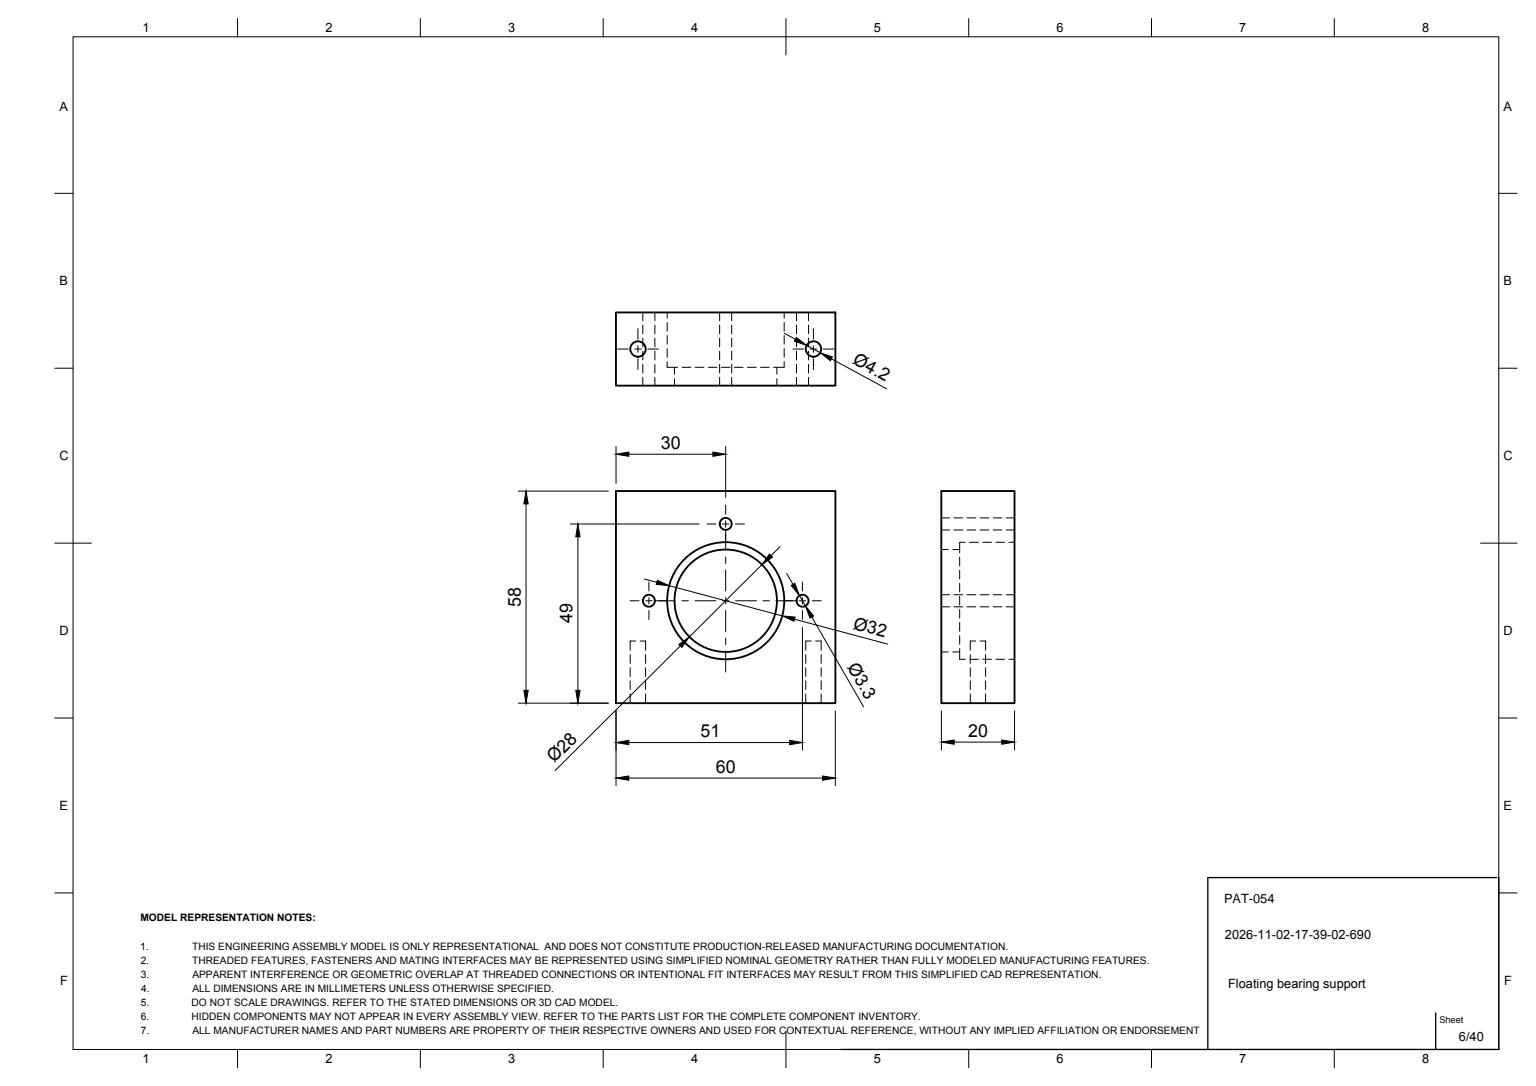
ISO-10303-21;
HEADER;
/* Generated by software containing ST-Developer
 * from STEP Tools, Inc. (www.steptools.com) 
 */

FILE_DESCRIPTION(
/* description */ ('PAT-054'),
/* implementation_level */ '2;1');

FILE_NAME(
/* name */ 'Floating bearing support.step',
/* time_stamp */ '2026-10-29T16:38:13-07:00',
/* author */ (''),
/* organization */ (''),
/* preprocessor_version */ 'ST-DEVELOPER v20.2',
/* originating_system */ 'Autodesk Translation Framework v15.17.0.0',
/* authorisation */ '');

FILE_SCHEMA (('AUTOMOTIVE_DESIGN { 1 0 10303 214 3 1 1 }'));
ENDSEC;

DATA;
#10=MECHANICAL_DESIGN_GEOMETRIC_PRESENTATION_REPRESENTATION('',(#901),#33981);
#813=SHAPE_REPRESENTATION_RELATIONSHIP('SRR','None',#34186,#857);
#857=ADVANCED_BREP_SHAPE_REPRESENTATION('',(#960),#33934);
#901=STYLED_ITEM('',(#34517),#960);
#960=MANIFOLD_SOLID_BREP('Body1',#13012);
#1064=FACE_BOUND('',#2399,.T.);
#1065=FACE_BOUND('',#2407,.T.);
#1066=FACE_BOUND('',#2408,.T.);
#1067=FACE_BOUND('',#2409,.T.);
#1068=FACE_BOUND('',#2410,.T.);
#1069=FACE_BOUND('',#2413,.T.);
#1070=FACE_BOUND('',#2414,.T.);
#1071=FACE_BOUND('',#2415,.T.);
#1072=FACE_BOUND('',#2416,.T.);
#1073=FACE_BOUND('',#2419,.T.);
#1074=FACE_BOUND('',#2420,.T.);
#1244=PLANE('',#13676);
#1245=PLANE('',#13683);
#1246=PLANE('',#13687);
#1247=PLANE('',#13688);
#1248=PLANE('',#13689);
#1249=PLANE('',#13690);
#1250=PLANE('',#13691);
#1251=PLANE('',#13692);
#1252=PLANE('',#13693);
#1619=FACE_OUTER_BOUND('',#2394,.T.);
#1620=FACE_OUTER_BOUND('',#2395,.T.);
#1621=FACE_OUTER_BOUND('',#2396,.T.);
#1622=FACE_OUTER_BOUND('',#2397,.T.);
#1623=FACE_OUTER_BOUND('',#2398,.T.);
#1624=FACE_OUTER_BOUND('',#2400,.T.);
#1625=FACE_OUTER_BOUND('',#2401,.T.);
#1626=FACE_OUTER_BOUND('',#2402,.T.);
#1627=FACE_OUTER_BOUND('',#2403,.T.);
#1628=FACE_OUTER_BOUND('',#2404,.T.);
#1629=FACE_OUTER_BOUND('',#2405,.T.);
#1630=FACE_OUTER_BOUND('',#2406,.T.);
#1631=FACE_OUTER_BOUND('',#2411,.T.);
#1632=FACE_OUTER_BOUND('',#2412,.T.);
#1633=FACE_OUTER_BOUND('',#2417,.T.);
#1634=FACE_OUTER_BOUND('',#2418,.T.);
#2394=EDGE_LOOP('',(#8705,#8706,#8707,#8708));
#2395=EDGE_LOOP('',(#8709,#8710,#8711,#8712));
#2396=EDGE_LOOP('',(#8713,#8714,#8715,#8716));
#2397=EDGE_LOOP('',(#8717,#8718,#8719,#8720));
#2398=EDGE_LOOP('',(#8721));
#2399=EDGE_LOOP('',(#8722));
#2400=EDGE_LOOP('',(#8723,#8724,#8725,#8726));
#2401=EDGE_LOOP('',(#8727,#8728,#8729,#8730));
#2402=EDGE_LOOP('',(#8731));
#2403=EDGE_LOOP('',(#8732,#8733,#8734,#8735));
#2404=EDGE_LOOP('',(#8736));
#2405=EDGE_LOOP('',(#8737,#8738,#8739,#8740));
#2406=EDGE_LOOP('',(#8741,#8742,#8743,#8744));
#2407=EDGE_LOOP('',(#8745));
#2408=EDGE_LOOP('',(#8746));
#2409=EDGE_LOOP('',(#8747));
#2410=EDGE_LOOP('',(#8748));
#2411=EDGE_LOOP('',(#8749,#8750,#8751,#8752));
#2412=EDGE_LOOP('',(#8753,#8754,#8755,#8756));
#2413=EDGE_LOOP('',(#8757));
#2414=EDGE_LOOP('',(#8758));
#2415=EDGE_LOOP('',(#8759));
#2416=EDGE_LOOP('',(#8760));
#2417=EDGE_LOOP('',(#8761,#8762,#8763,#8764));
#2418=EDGE_LOOP('',(#8765,#8766,#8767,#8768));
#2419=EDGE_LOOP('',(#8769));
#2420=EDGE_LOOP('',(#8770));
#3289=LINE('',#18719,#4223);
#3290=LINE('',#18725,#4224);
#3291=LINE('',#18731,#4225);
#3292=LINE('',#18737,#4226);
#3293=LINE('',#18744,#4227);
#3294=LINE('',#18750,#4228);
#3295=LINE('',#18757,#4229);
#3296=LINE('',#18763,#4230);
#3297=LINE('',#18765,#4231);
#3298=LINE('',#18767,#4232);
#3299=LINE('',#18768,#4233);
#3300=LINE('',#18771,#4234);
#3301=LINE('',#18773,#4235);
#3302=LINE('',#18774,#4236);
#3303=LINE('',#18777,#4237);
#3304=LINE('',#18779,#4238);
#3305=LINE('',#18780,#4239);
#3306=LINE('',#18782,#4240);
#3307=LINE('',#18783,#4241);
#4223=VECTOR('',#15156,0.165);
#4224=VECTOR('',#15163,0.165);
#4225=VECTOR('',#15170,0.165);
#4226=VECTOR('',#15177,1.6);
#4227=VECTOR('',#15186,1.4);
#4228=VECTOR('',#15193,0.21);
#4229=VECTOR('',#15202,0.21);
#4230=VECTOR('',#15209,1.);
#4231=VECTOR('',#15210,1.);
#4232=VECTOR('',#15211,1.);
#4233=VECTOR('',#15212,1.);
#4234=VECTOR('',#15215,1.);
#4235=VECTOR('',#15216,1.);
#4236=VECTOR('',#15217,1.);
#4237=VECTOR('',#15220,1.);
#4238=VECTOR('',#15221,1.);
#4239=VECTOR('',#15222,1.);
#4240=VECTOR('',#15225,1.);
#4241=VECTOR('',#15226,1.);
#5161=CIRCLE('',#13665,0.165);
#5162=CIRCLE('',#13666,0.165);
#5163=CIRCLE('',#13668,0.165);
#5164=CIRCLE('',#13669,0.165);
#5165=CIRCLE('',#13671,0.165);
#5166=CIRCLE('',#13672,0.165);
#5167=CIRCLE('',#13674,1.6);
#5168=CIRCLE('',#13675,1.6);
#5169=CIRCLE('',#13677,1.4);
#5170=CIRCLE('',#13679,1.4);
#5171=CIRCLE('',#13681,0.21);
#5172=CIRCLE('',#13682,0.21);
#5173=CIRCLE('',#13685,0.21);
#5174=CIRCLE('',#13686,0.21);
#5642=VERTEX_POINT('',#18716);
#5643=VERTEX_POINT('',#18718);
#5644=VERTEX_POINT('',#18722);
#5645=VERTEX_POINT('',#18724);
#5646=VERTEX_POINT('',#18728);
#5647=VERTEX_POINT('',#18730);
#5648=VERTEX_POINT('',#18734);
#5649=VERTEX_POINT('',#18736);
#5650=VERTEX_POINT('',#18740);
#5651=VERTEX_POINT('',#18743);
#5652=VERTEX_POINT('',#18747);
#5653=VERTEX_POINT('',#18749);
#5654=VERTEX_POINT('',#18754);
#5655=VERTEX_POINT('',#18756);
#5656=VERTEX_POINT('',#18761);
#5657=VERTEX_POINT('',#18762);
#5658=VERTEX_POINT('',#18764);
#5659=VERTEX_POINT('',#18766);
#5660=VERTEX_POINT('',#18770);
#5661=VERTEX_POINT('',#18772);
#5662=VERTEX_POINT('',#18776);
#5663=VERTEX_POINT('',#18778);
#6852=EDGE_CURVE('',#5642,#5642,#5161,.T.);
#6853=EDGE_CURVE('',#5642,#5643,#3289,.T.);
#6854=EDGE_CURVE('',#5643,#5643,#5162,.T.);
#6855=EDGE_CURVE('',#5644,#5644,#5163,.T.);
#6856=EDGE_CURVE('',#5644,#5645,#3290,.T.);
#6857=EDGE_CURVE('',#5645,#5645,#5164,.T.);
#6858=EDGE_CURVE('',#5646,#5646,#5165,.T.);
#6859=EDGE_CURVE('',#5646,#5647,#3291,.T.);
#6860=EDGE_CURVE('',#5647,#5647,#5166,.T.);
#6861=EDGE_CURVE('',#5648,#5648,#5167,.T.);
#6862=EDGE_CURVE('',#5648,#5649,#3292,.T.);
#6863=EDGE_CURVE('',#5649,#5649,#5168,.T.);
#6864=EDGE_CURVE('',#5650,#5650,#5169,.T.);
#6865=EDGE_CURVE('',#5650,#5651,#3293,.T.);
#6866=EDGE_CURVE('',#5651,#5651,#5170,.T.);
#6867=EDGE_CURVE('',#5652,#5652,#5171,.T.);
#6868=EDGE_CURVE('',#5652,#5653,#3294,.T.);
#6869=EDGE_CURVE('',#5653,#5653,#5172,.T.);
#6870=EDGE_CURVE('',#5654,#5654,#5173,.T.);
#6871=EDGE_CURVE('',#5654,#5655,#3295,.T.);
#6872=EDGE_CURVE('',#5655,#5655,#5174,.T.);
#6873=EDGE_CURVE('',#5656,#5657,#3296,.T.);
#6874=EDGE_CURVE('',#5657,#5658,#3297,.T.);
#6875=EDGE_CURVE('',#5659,#5658,#3298,.T.);
#6876=EDGE_CURVE('',#5656,#5659,#3299,.T.);
#6877=EDGE_CURVE('',#5660,#5656,#3300,.T.);
#6878=EDGE_CURVE('',#5661,#5659,#3301,.T.);
#6879=EDGE_CURVE('',#5660,#5661,#3302,.T.);
#6880=EDGE_CURVE('',#5662,#5660,#3303,.T.);
#6881=EDGE_CURVE('',#5663,#5661,#3304,.T.);
#6882=EDGE_CURVE('',#5662,#5663,#3305,.T.);
#6883=EDGE_CURVE('',#5657,#5662,#3306,.T.);
#6884=EDGE_CURVE('',#5658,#5663,#3307,.T.);
#8705=ORIENTED_EDGE('',*,*,#6852,.F.);
#8706=ORIENTED_EDGE('',*,*,#6853,.T.);
#8707=ORIENTED_EDGE('',*,*,#6854,.F.);
#8708=ORIENTED_EDGE('',*,*,#6853,.F.);
#8709=ORIENTED_EDGE('',*,*,#6855,.F.);
#8710=ORIENTED_EDGE('',*,*,#6856,.T.);
#8711=ORIENTED_EDGE('',*,*,#6857,.F.);
#8712=ORIENTED_EDGE('',*,*,#6856,.F.);
#8713=ORIENTED_EDGE('',*,*,#6858,.F.);
#8714=ORIENTED_EDGE('',*,*,#6859,.T.);
#8715=ORIENTED_EDGE('',*,*,#6860,.F.);
#8716=ORIENTED_EDGE('',*,*,#6859,.F.);
#8717=ORIENTED_EDGE('',*,*,#6861,.F.);
#8718=ORIENTED_EDGE('',*,*,#6862,.T.);
#8719=ORIENTED_EDGE('',*,*,#6863,.T.);
#8720=ORIENTED_EDGE('',*,*,#6862,.F.);
#8721=ORIENTED_EDGE('',*,*,#6863,.F.);
#8722=ORIENTED_EDGE('',*,*,#6864,.F.);
#8723=ORIENTED_EDGE('',*,*,#6864,.T.);
#8724=ORIENTED_EDGE('',*,*,#6865,.T.);
#8725=ORIENTED_EDGE('',*,*,#6866,.F.);
#8726=ORIENTED_EDGE('',*,*,#6865,.F.);
#8727=ORIENTED_EDGE('',*,*,#6867,.F.);
#8728=ORIENTED_EDGE('',*,*,#6868,.T.);
#8729=ORIENTED_EDGE('',*,*,#6869,.T.);
#8730=ORIENTED_EDGE('',*,*,#6868,.F.);
#8731=ORIENTED_EDGE('',*,*,#6869,.F.);
#8732=ORIENTED_EDGE('',*,*,#6870,.F.);
#8733=ORIENTED_EDGE('',*,*,#6871,.T.);
#8734=ORIENTED_EDGE('',*,*,#6872,.T.);
#8735=ORIENTED_EDGE('',*,*,#6871,.F.);
#8736=ORIENTED_EDGE('',*,*,#6872,.F.);
#8737=ORIENTED_EDGE('',*,*,#6873,.T.);
#8738=ORIENTED_EDGE('',*,*,#6874,.T.);
#8739=ORIENTED_EDGE('',*,*,#6875,.F.);
#8740=ORIENTED_EDGE('',*,*,#6876,.F.);
#8741=ORIENTED_EDGE('',*,*,#6877,.T.);
#8742=ORIENTED_EDGE('',*,*,#6876,.T.);
#8743=ORIENTED_EDGE('',*,*,#6878,.F.);
#8744=ORIENTED_EDGE('',*,*,#6879,.F.);
#8745=ORIENTED_EDGE('',*,*,#6854,.T.);
#8746=ORIENTED_EDGE('',*,*,#6857,.T.);
#8747=ORIENTED_EDGE('',*,*,#6860,.T.);
#8748=ORIENTED_EDGE('',*,*,#6866,.T.);
#8749=ORIENTED_EDGE('',*,*,#6880,.T.);
#8750=ORIENTED_EDGE('',*,*,#6879,.T.);
#8751=ORIENTED_EDGE('',*,*,#6881,.F.);
#8752=ORIENTED_EDGE('',*,*,#6882,.F.);
#8753=ORIENTED_EDGE('',*,*,#6883,.T.);
#8754=ORIENTED_EDGE('',*,*,#6882,.T.);
#8755=ORIENTED_EDGE('',*,*,#6884,.F.);
#8756=ORIENTED_EDGE('',*,*,#6874,.F.);
#8757=ORIENTED_EDGE('',*,*,#6852,.T.);
#8758=ORIENTED_EDGE('',*,*,#6855,.T.);
#8759=ORIENTED_EDGE('',*,*,#6858,.T.);
#8760=ORIENTED_EDGE('',*,*,#6861,.T.);
#8761=ORIENTED_EDGE('',*,*,#6884,.T.);
#8762=ORIENTED_EDGE('',*,*,#6881,.T.);
#8763=ORIENTED_EDGE('',*,*,#6878,.T.);
#8764=ORIENTED_EDGE('',*,*,#6875,.T.);
#8765=ORIENTED_EDGE('',*,*,#6883,.F.);
#8766=ORIENTED_EDGE('',*,*,#6873,.F.);
#8767=ORIENTED_EDGE('',*,*,#6877,.F.);
#8768=ORIENTED_EDGE('',*,*,#6880,.F.);
#8769=ORIENTED_EDGE('',*,*,#6867,.T.);
#8770=ORIENTED_EDGE('',*,*,#6870,.T.);
#12007=CYLINDRICAL_SURFACE('',#13664,0.165);
#12008=CYLINDRICAL_SURFACE('',#13667,0.165);
#12009=CYLINDRICAL_SURFACE('',#13670,0.165);
#12010=CYLINDRICAL_SURFACE('',#13673,1.6);
#12011=CYLINDRICAL_SURFACE('',#13678,1.4);
#12012=CYLINDRICAL_SURFACE('',#13680,0.21);
#12013=CYLINDRICAL_SURFACE('',#13684,0.21);
#12331=ADVANCED_FACE('',(#1619),#12007,.F.);
#12332=ADVANCED_FACE('',(#1620),#12008,.F.);
#12333=ADVANCED_FACE('',(#1621),#12009,.F.);
#12334=ADVANCED_FACE('',(#1622),#12010,.F.);
#12335=ADVANCED_FACE('',(#1623,#1064),#1244,.F.);
#12336=ADVANCED_FACE('',(#1624),#12011,.F.);
#12337=ADVANCED_FACE('',(#1625),#12012,.F.);
#12338=ADVANCED_FACE('',(#1626),#1245,.F.);
#12339=ADVANCED_FACE('',(#1627),#12013,.F.);
#12340=ADVANCED_FACE('',(#1628),#1246,.F.);
#12341=ADVANCED_FACE('',(#1629),#1247,.T.);
#12342=ADVANCED_FACE('',(#1630,#1065,#1066,#1067,#1068),#1248,.T.);
#12343=ADVANCED_FACE('',(#1631),#1249,.T.);
#12344=ADVANCED_FACE('',(#1632,#1069,#1070,#1071,#1072),#1250,.T.);
#12345=ADVANCED_FACE('',(#1633),#1251,.T.);
#12346=ADVANCED_FACE('',(#1634,#1073,#1074),#1252,.F.);
#13012=CLOSED_SHELL('',(#12331,#12332,#12333,#12334,#12335,#12336,#12337,
#12338,#12339,#12340,#12341,#12342,#12343,#12344,#12345,#12346));
#13663=AXIS2_PLACEMENT_3D('',#18714,#15150,#15151);
#13664=AXIS2_PLACEMENT_3D('',#18715,#15152,#15153);
#13665=AXIS2_PLACEMENT_3D('',#18717,#15154,#15155);
#13666=AXIS2_PLACEMENT_3D('',#18720,#15157,#15158);
#13667=AXIS2_PLACEMENT_3D('',#18721,#15159,#15160);
#13668=AXIS2_PLACEMENT_3D('',#18723,#15161,#15162);
#13669=AXIS2_PLACEMENT_3D('',#18726,#15164,#15165);
#13670=AXIS2_PLACEMENT_3D('',#18727,#15166,#15167);
#13671=AXIS2_PLACEMENT_3D('',#18729,#15168,#15169);
#13672=AXIS2_PLACEMENT_3D('',#18732,#15171,#15172);
#13673=AXIS2_PLACEMENT_3D('',#18733,#15173,#15174);
#13674=AXIS2_PLACEMENT_3D('',#18735,#15175,#15176);
#13675=AXIS2_PLACEMENT_3D('',#18738,#15178,#15179);
#13676=AXIS2_PLACEMENT_3D('',#18739,#15180,#15181);
#13677=AXIS2_PLACEMENT_3D('',#18741,#15182,#15183);
#13678=AXIS2_PLACEMENT_3D('',#18742,#15184,#15185);
#13679=AXIS2_PLACEMENT_3D('',#18745,#15187,#15188);
#13680=AXIS2_PLACEMENT_3D('',#18746,#15189,#15190);
#13681=AXIS2_PLACEMENT_3D('',#18748,#15191,#15192);
#13682=AXIS2_PLACEMENT_3D('',#18751,#15194,#15195);
#13683=AXIS2_PLACEMENT_3D('',#18752,#15196,#15197);
#13684=AXIS2_PLACEMENT_3D('',#18753,#15198,#15199);
#13685=AXIS2_PLACEMENT_3D('',#18755,#15200,#15201);
#13686=AXIS2_PLACEMENT_3D('',#18758,#15203,#15204);
#13687=AXIS2_PLACEMENT_3D('',#18759,#15205,#15206);
#13688=AXIS2_PLACEMENT_3D('',#18760,#15207,#15208);
#13689=AXIS2_PLACEMENT_3D('',#18769,#15213,#15214);
#13690=AXIS2_PLACEMENT_3D('',#18775,#15218,#15219);
#13691=AXIS2_PLACEMENT_3D('',#18781,#15223,#15224);
#13692=AXIS2_PLACEMENT_3D('',#18784,#15227,#15228);
#13693=AXIS2_PLACEMENT_3D('',#18785,#15229,#15230);
#15150=DIRECTION('axis',(0.,0.,1.));
#15151=DIRECTION('refdir',(1.,0.,0.));
#15152=DIRECTION('center_axis',(1.,0.,0.));
#15153=DIRECTION('ref_axis',(0.,0.,-1.));
#15154=DIRECTION('center_axis',(1.,0.,0.));
#15155=DIRECTION('ref_axis',(0.,0.,-1.));
#15156=DIRECTION('',(1.,0.,0.));
#15157=DIRECTION('center_axis',(-1.,0.,0.));
#15158=DIRECTION('ref_axis',(0.,0.,-1.));
#15159=DIRECTION('center_axis',(1.,0.,0.));
#15160=DIRECTION('ref_axis',(0.,0.,-1.));
#15161=DIRECTION('center_axis',(1.,0.,0.));
#15162=DIRECTION('ref_axis',(0.,0.,-1.));
#15163=DIRECTION('',(1.,0.,0.));
#15164=DIRECTION('center_axis',(-1.,0.,0.));
#15165=DIRECTION('ref_axis',(0.,0.,-1.));
#15166=DIRECTION('center_axis',(1.,0.,0.));
#15167=DIRECTION('ref_axis',(0.,0.,-1.));
#15168=DIRECTION('center_axis',(1.,0.,0.));
#15169=DIRECTION('ref_axis',(0.,0.,-1.));
#15170=DIRECTION('',(1.,0.,0.));
#15171=DIRECTION('center_axis',(-1.,0.,0.));
#15172=DIRECTION('ref_axis',(0.,0.,-1.));
#15173=DIRECTION('center_axis',(1.,0.,0.));
#15174=DIRECTION('ref_axis',(0.,0.,-1.));
#15175=DIRECTION('center_axis',(1.,0.,0.));
#15176=DIRECTION('ref_axis',(0.,0.,-1.));
#15177=DIRECTION('',(1.,0.,0.));
#15178=DIRECTION('center_axis',(1.,0.,0.));
#15179=DIRECTION('ref_axis',(0.,0.,-1.));
#15180=DIRECTION('center_axis',(1.,0.,0.));
#15181=DIRECTION('ref_axis',(0.,0.,-1.));
#15182=DIRECTION('center_axis',(-1.,0.,0.));
#15183=DIRECTION('ref_axis',(0.,0.,-1.));
#15184=DIRECTION('center_axis',(1.,0.,0.));
#15185=DIRECTION('ref_axis',(0.,0.,-1.));
#15186=DIRECTION('',(1.,0.,0.));
#15187=DIRECTION('center_axis',(-1.,0.,0.));
#15188=DIRECTION('ref_axis',(0.,0.,-1.));
#15189=DIRECTION('center_axis',(0.,0.,1.));
#15190=DIRECTION('ref_axis',(1.,0.,0.));
#15191=DIRECTION('center_axis',(0.,0.,1.));
#15192=DIRECTION('ref_axis',(1.,0.,0.));
#15193=DIRECTION('',(0.,0.,1.));
#15194=DIRECTION('center_axis',(0.,0.,1.));
#15195=DIRECTION('ref_axis',(1.,0.,0.));
#15196=DIRECTION('center_axis',(0.,0.,1.));
#15197=DIRECTION('ref_axis',(1.,0.,0.));
#15198=DIRECTION('center_axis',(0.,0.,1.));
#15199=DIRECTION('ref_axis',(1.,0.,0.));
#15200=DIRECTION('center_axis',(0.,0.,1.));
#15201=DIRECTION('ref_axis',(1.,0.,0.));
#15202=DIRECTION('',(0.,0.,1.));
#15203=DIRECTION('center_axis',(0.,0.,1.));
#15204=DIRECTION('ref_axis',(1.,0.,0.));
#15205=DIRECTION('center_axis',(0.,0.,1.));
#15206=DIRECTION('ref_axis',(1.,0.,0.));
#15207=DIRECTION('center_axis',(0.,1.,0.));
#15208=DIRECTION('ref_axis',(-1.,0.,0.));
#15209=DIRECTION('',(-1.,0.,0.));
#15210=DIRECTION('',(0.,0.,1.));
#15211=DIRECTION('',(-1.,0.,0.));
#15212=DIRECTION('',(0.,0.,1.));
#15213=DIRECTION('center_axis',(1.,0.,0.));
#15214=DIRECTION('ref_axis',(0.,1.,0.));
#15215=DIRECTION('',(0.,1.,0.));
#15216=DIRECTION('',(0.,1.,0.));
#15217=DIRECTION('',(0.,0.,1.));
#15218=DIRECTION('center_axis',(0.,-1.,0.));
#15219=DIRECTION('ref_axis',(1.,0.,0.));
#15220=DIRECTION('',(1.,0.,0.));
#15221=DIRECTION('',(1.,0.,0.));
#15222=DIRECTION('',(0.,0.,1.));
#15223=DIRECTION('center_axis',(-1.,0.,0.));
#15224=DIRECTION('ref_axis',(0.,-1.,0.));
#15225=DIRECTION('',(0.,-1.,0.));
#15226=DIRECTION('',(0.,-1.,0.));
#15227=DIRECTION('center_axis',(0.,0.,1.));
#15228=DIRECTION('ref_axis',(1.,0.,0.));
#15229=DIRECTION('center_axis',(0.,0.,1.));
#15230=DIRECTION('ref_axis',(1.,0.,0.));
#18714=CARTESIAN_POINT('',(0.,0.,0.));
#18715=CARTESIAN_POINT('Origin',(1.9,-2.1,4.));
#18716=CARTESIAN_POINT('',(2.,-2.1,4.165));
#18717=CARTESIAN_POINT('Origin',(2.,-2.1,4.));
#18718=CARTESIAN_POINT('',(4.,-2.1,4.165));
#18719=CARTESIAN_POINT('',(1.9,-2.1,4.165));
#18720=CARTESIAN_POINT('Origin',(4.,-2.1,4.));
#18721=CARTESIAN_POINT('Origin',(1.9,2.1,4.));
#18722=CARTESIAN_POINT('',(2.,2.1,4.165));
#18723=CARTESIAN_POINT('Origin',(2.,2.1,4.));
#18724=CARTESIAN_POINT('',(4.,2.1,4.165));
#18725=CARTESIAN_POINT('',(1.9,2.1,4.165));
#18726=CARTESIAN_POINT('Origin',(4.,2.1,4.));
#18727=CARTESIAN_POINT('Origin',(1.9,0.,6.1));
#18728=CARTESIAN_POINT('',(2.,-2.02066721859313E-17,6.265));
#18729=CARTESIAN_POINT('Origin',(2.,0.,6.1));
#18730=CARTESIAN_POINT('',(4.,2.02066721859313E-17,6.265));
#18731=CARTESIAN_POINT('',(1.9,-2.02066721859313E-17,6.265));
#18732=CARTESIAN_POINT('Origin',(4.,0.,6.1));
#18733=CARTESIAN_POINT('Origin',(1.9,0.,4.));
#18734=CARTESIAN_POINT('',(2.,-1.95943487863577E-16,5.6));
#18735=CARTESIAN_POINT('Origin',(2.,0.,4.));
#18736=CARTESIAN_POINT('',(3.5,-1.95943487863577E-16,5.6));
#18737=CARTESIAN_POINT('',(1.9,-1.95943487863577E-16,5.6));
#18738=CARTESIAN_POINT('Origin',(3.5,0.,4.));
#18739=CARTESIAN_POINT('Origin',(3.5,0.,4.));
#18740=CARTESIAN_POINT('',(3.5,1.71450551880629E-16,5.4));
#18741=CARTESIAN_POINT('Origin',(3.5,0.,4.));
#18742=CARTESIAN_POINT('Origin',(1.9,0.,4.));
#18743=CARTESIAN_POINT('',(4.,1.71450551880629E-16,5.4));
#18744=CARTESIAN_POINT('',(1.9,-1.71450551880629E-16,5.4));
#18745=CARTESIAN_POINT('Origin',(4.,0.,4.));
#18746=CARTESIAN_POINT('Origin',(3.,-2.4,1.1));
#18747=CARTESIAN_POINT('',(2.79,-2.4,1.2));
#18748=CARTESIAN_POINT('Origin',(3.,-2.4,1.2));
#18749=CARTESIAN_POINT('',(2.79,-2.4,2.9));
#18750=CARTESIAN_POINT('',(2.79,-2.4,1.1));
#18751=CARTESIAN_POINT('Origin',(3.,-2.4,2.9));
#18752=CARTESIAN_POINT('Origin',(3.,-2.4,2.9));
#18753=CARTESIAN_POINT('Origin',(3.,2.4,1.1));
#18754=CARTESIAN_POINT('',(2.79,2.4,1.2));
#18755=CARTESIAN_POINT('Origin',(3.,2.4,1.2));
#18756=CARTESIAN_POINT('',(2.79,2.4,2.9));
#18757=CARTESIAN_POINT('',(2.79,2.4,1.1));
#18758=CARTESIAN_POINT('Origin',(3.,2.4,2.9));
#18759=CARTESIAN_POINT('Origin',(3.,2.4,2.9));
#18760=CARTESIAN_POINT('Origin',(4.,3.,1.2));
#18761=CARTESIAN_POINT('',(4.,3.,1.2));
#18762=CARTESIAN_POINT('',(2.,3.,1.2));
#18763=CARTESIAN_POINT('',(4.,3.,1.2));
#18764=CARTESIAN_POINT('',(2.,3.,7.));
#18765=CARTESIAN_POINT('',(2.,3.,1.2));
#18766=CARTESIAN_POINT('',(4.,3.,7.));
#18767=CARTESIAN_POINT('',(4.,3.,7.));
#18768=CARTESIAN_POINT('',(4.,3.,1.2));
#18769=CARTESIAN_POINT('Origin',(4.,-3.,1.2));
#18770=CARTESIAN_POINT('',(4.,-3.,1.2));
#18771=CARTESIAN_POINT('',(4.,-3.,1.2));
#18772=CARTESIAN_POINT('',(4.,-3.,7.));
#18773=CARTESIAN_POINT('',(4.,-3.,7.));
#18774=CARTESIAN_POINT('',(4.,-3.,1.2));
#18775=CARTESIAN_POINT('Origin',(2.,-3.,1.2));
#18776=CARTESIAN_POINT('',(2.,-3.,1.2));
#18777=CARTESIAN_POINT('',(2.,-3.,1.2));
#18778=CARTESIAN_POINT('',(2.,-3.,7.));
#18779=CARTESIAN_POINT('',(2.,-3.,7.));
#18780=CARTESIAN_POINT('',(2.,-3.,1.2));
#18781=CARTESIAN_POINT('Origin',(2.,3.,1.2));
#18782=CARTESIAN_POINT('',(2.,3.,1.2));
#18783=CARTESIAN_POINT('',(2.,3.,7.));
#18784=CARTESIAN_POINT('Origin',(3.,0.,7.));
#18785=CARTESIAN_POINT('Origin',(3.,0.,1.2));
#33882=UNCERTAINTY_MEASURE_WITH_UNIT(LENGTH_MEASURE(0.001),#33982,
'DISTANCE_ACCURACY_VALUE',
'Maximum model space distance between geometric entities at asserted c
onnectivities');
#33929=UNCERTAINTY_MEASURE_WITH_UNIT(LENGTH_MEASURE(0.001),#33982,
'DISTANCE_ACCURACY_VALUE',
'Maximum model space distance between geometric entities at asserted c
onnectivities');
#33934=(
GEOMETRIC_REPRESENTATION_CONTEXT(3)
GLOBAL_UNCERTAINTY_ASSIGNED_CONTEXT((#33882))
GLOBAL_UNIT_ASSIGNED_CONTEXT((#33982,#33984,#33985))
REPRESENTATION_CONTEXT('','3D')
);
#33981=(
GEOMETRIC_REPRESENTATION_CONTEXT(3)
GLOBAL_UNCERTAINTY_ASSIGNED_CONTEXT((#33929))
GLOBAL_UNIT_ASSIGNED_CONTEXT((#33982,#33984,#33985))
REPRESENTATION_CONTEXT('','3D')
);
#33982=(
LENGTH_UNIT()
NAMED_UNIT(*)
SI_UNIT(.CENTI.,.METRE.)
);
#33984=(
NAMED_UNIT(*)
PLANE_ANGLE_UNIT()
SI_UNIT($,.RADIAN.)
);
#33985=(
NAMED_UNIT(*)
SI_UNIT($,.STERADIAN.)
SOLID_ANGLE_UNIT()
);
#33990=SHAPE_DEFINITION_REPRESENTATION(#34041,#34186);
#34041=PRODUCT_DEFINITION_SHAPE('',$,#34238);
#34186=SHAPE_REPRESENTATION('',(#13663),#33934);
#34233=PRODUCT_DEFINITION_CONTEXT('part definition',#34388,'design');
#34238=PRODUCT_DEFINITION('Floating bearing support',
'Floating bearing support',#34289,#34233);
#34289=PRODUCT_DEFINITION_FORMATION('',$,#34394);
#34388=APPLICATION_CONTEXT(
'Core Data for Automotive Mechanical Design Process');
#34389=PRODUCT_CONTEXT('part definition',#34388,'mechanical');
#34394=PRODUCT('Floating bearing support','Floating bearing support',
'Floating bearing support',(#34389));
#34511=COLOUR_RGB('Grey',0.48,0.52,0.57);
#34512=FILL_AREA_STYLE_COLOUR('',#34511);
#34513=FILL_AREA_STYLE('',(#34512));
#34514=SURFACE_STYLE_FILL_AREA(#34513);
#34515=SURFACE_SIDE_STYLE('',(#34514));
#34516=SURFACE_STYLE_USAGE(.BOTH.,#34515);
#34517=PRESENTATION_STYLE_ASSIGNMENT((#34516));
ENDSEC;
END-ISO-10303-21;
